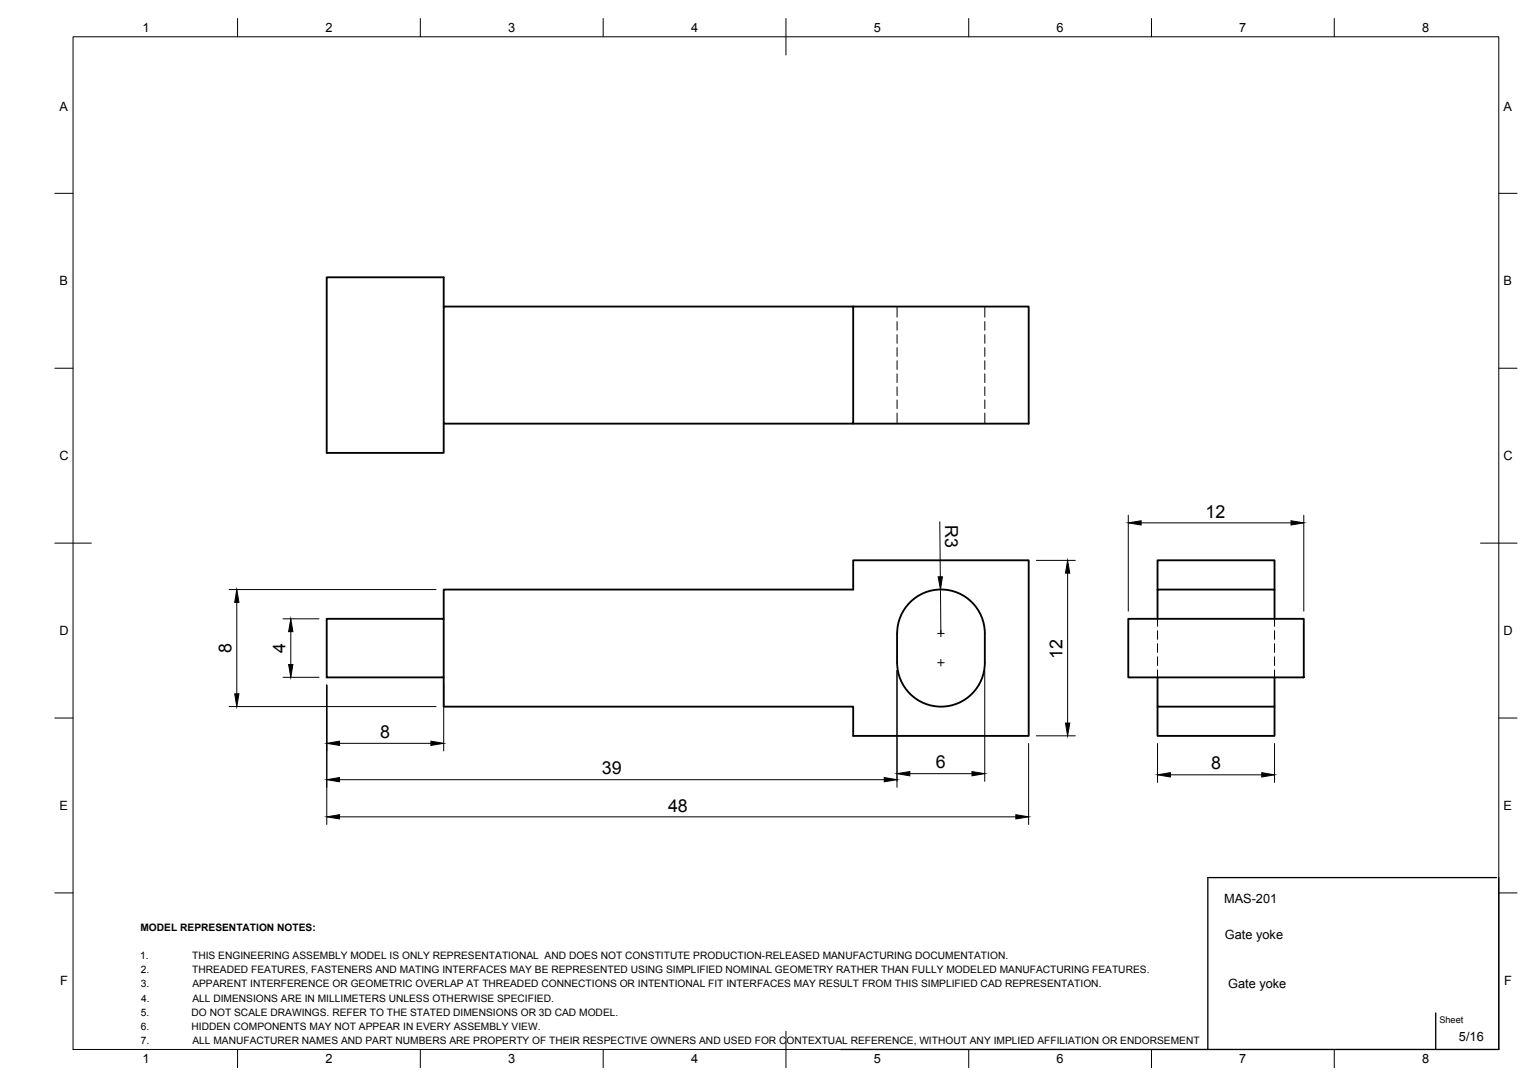
ISO-10303-21;
HEADER;
/* Generated by software containing ST-Developer
 * from STEP Tools, Inc. (www.steptools.com) 
 */

FILE_DESCRIPTION(
/* description */ ('Independent manual two-gate roller-track escapement for nominal30mm d
iameter20mm wide feed rollers. Opposed gates are driven by native capt
ured pin-slot loops with positive curved-slot travel stops at\X\B116de
g. Repeated gate/pin/washer/clip instances, adapted native common bear
ing families, full retaining lips and rotating polymer grip. External 
workpieces, gravity feeder/incline and mount anchors outside assembly.
 No powered-feed compatibility, impact, capacity, safety, force, wear 
or life rating.'),
/* implementation_level */ '2;1');

FILE_NAME(
/* name */ 'Gate yoke.step',
/* time_stamp */ '2026-11-08T18:43:23-08:00',
/* author */ (''),
/* organization */ (''),
/* preprocessor_version */ 'ST-DEVELOPER v20.2',
/* originating_system */ 'Autodesk Translation Framework v15.17.0.0',
/* authorisation */ '');

FILE_SCHEMA (('AUTOMOTIVE_DESIGN { 1 0 10303 214 3 1 1 }'));
ENDSEC;

DATA;
#10=MECHANICAL_DESIGN_GEOMETRIC_PRESENTATION_REPRESENTATION('',(#458),#19863);
#420=SHAPE_REPRESENTATION_RELATIONSHIP('SRR','None',#19938,#439);
#439=ADVANCED_BREP_SHAPE_REPRESENTATION('',(#477),#19847);
#458=STYLED_ITEM('',(#20041),#477);
#477=MANIFOLD_SOLID_BREP('Body1',#6427);
#774=LINE('',#15657,#1239);
#775=LINE('',#15659,#1240);
#776=LINE('',#15661,#1241);
#777=LINE('',#15662,#1242);
#778=LINE('',#15667,#1243);
#779=LINE('',#15671,#1244);
#780=LINE('',#15673,#1245);
#781=LINE('',#15674,#1246);
#782=LINE('',#15681,#1247);
#783=LINE('',#15683,#1248);
#784=LINE('',#15685,#1249);
#785=LINE('',#15686,#1250);
#786=LINE('',#15690,#1251);
#787=LINE('',#15692,#1252);
#788=LINE('',#15694,#1253);
#789=LINE('',#15695,#1254);
#790=LINE('',#15698,#1255);
#791=LINE('',#15700,#1256);
#792=LINE('',#15701,#1257);
#793=LINE('',#15703,#1258);
#794=LINE('',#15705,#1259);
#795=LINE('',#15706,#1260);
#796=LINE('',#15709,#1261);
#797=LINE('',#15710,#1262);
#798=LINE('',#15712,#1263);
#799=LINE('',#15713,#1264);
#800=LINE('',#15717,#1265);
#801=LINE('',#15719,#1266);
#802=LINE('',#15720,#1267);
#803=LINE('',#15723,#1268);
#804=LINE('',#15725,#1269);
#805=LINE('',#15726,#1270);
#806=LINE('',#15730,#1271);
#807=LINE('',#15731,#1272);
#808=LINE('',#15732,#1273);
#809=LINE('',#15736,#1274);
#810=LINE('',#15737,#1275);
#811=LINE('',#15738,#1276);
#812=LINE('',#15741,#1277);
#813=LINE('',#15743,#1278);
#814=LINE('',#15744,#1279);
#815=LINE('',#15748,#1280);
#816=LINE('',#15749,#1281);
#817=LINE('',#15751,#1282);
#818=LINE('',#15752,#1283);
#819=LINE('',#15755,#1284);
#820=LINE('',#15757,#1285);
#821=LINE('',#15758,#1286);
#822=LINE('',#15761,#1287);
#823=LINE('',#15762,#1288);
#824=LINE('',#15763,#1289);
#825=LINE('',#15765,#1290);
#1239=VECTOR('',#7968,10.);
#1240=VECTOR('',#7969,10.);
#1241=VECTOR('',#7970,10.);
#1242=VECTOR('',#7971,10.);
#1243=VECTOR('',#7976,10.);
#1244=VECTOR('',#7981,10.);
#1245=VECTOR('',#7982,10.);
#1246=VECTOR('',#7983,10.);
#1247=VECTOR('',#7992,10.);
#1248=VECTOR('',#7993,10.);
#1249=VECTOR('',#7994,10.);
#1250=VECTOR('',#7995,10.);
#1251=VECTOR('',#7998,10.);
#1252=VECTOR('',#7999,10.);
#1253=VECTOR('',#8000,10.);
#1254=VECTOR('',#8001,10.);
#1255=VECTOR('',#8004,10.);
#1256=VECTOR('',#8005,10.);
#1257=VECTOR('',#8006,10.);
#1258=VECTOR('',#8009,10.);
#1259=VECTOR('',#8010,10.);
#1260=VECTOR('',#8011,10.);
#1261=VECTOR('',#8014,10.);
#1262=VECTOR('',#8015,10.);
#1263=VECTOR('',#8018,10.);
#1264=VECTOR('',#8019,10.);
#1265=VECTOR('',#8024,10.);
#1266=VECTOR('',#8025,10.);
#1267=VECTOR('',#8026,10.);
#1268=VECTOR('',#8029,10.);
#1269=VECTOR('',#8030,10.);
#1270=VECTOR('',#8031,10.);
#1271=VECTOR('',#8034,10.);
#1272=VECTOR('',#8035,10.);
#1273=VECTOR('',#8036,10.);
#1274=VECTOR('',#8039,10.);
#1275=VECTOR('',#8040,10.);
#1276=VECTOR('',#8041,10.);
#1277=VECTOR('',#8044,10.);
#1278=VECTOR('',#8045,10.);
#1279=VECTOR('',#8046,10.);
#1280=VECTOR('',#8049,10.);
#1281=VECTOR('',#8050,10.);
#1282=VECTOR('',#8051,10.);
#1283=VECTOR('',#8052,10.);
#1284=VECTOR('',#8055,10.);
#1285=VECTOR('',#8056,10.);
#1286=VECTOR('',#8057,10.);
#1287=VECTOR('',#8060,10.);
#1288=VECTOR('',#8061,10.);
#1289=VECTOR('',#8062,10.);
#1290=VECTOR('',#8065,10.);
#1534=CYLINDRICAL_SURFACE('',#6901,3.);
#1535=CYLINDRICAL_SURFACE('',#6905,3.);
#1657=FACE_BOUND('',#2291,.T.);
#1658=FACE_BOUND('',#2294,.T.);
#1875=FACE_OUTER_BOUND('',#2274,.T.);
#1876=FACE_OUTER_BOUND('',#2275,.T.);
#1877=FACE_OUTER_BOUND('',#2276,.T.);
#1878=FACE_OUTER_BOUND('',#2277,.T.);
#1879=FACE_OUTER_BOUND('',#2278,.T.);
#1880=FACE_OUTER_BOUND('',#2279,.T.);
#1881=FACE_OUTER_BOUND('',#2280,.T.);
#1882=FACE_OUTER_BOUND('',#2281,.T.);
#1883=FACE_OUTER_BOUND('',#2282,.T.);
#1884=FACE_OUTER_BOUND('',#2283,.T.);
#1885=FACE_OUTER_BOUND('',#2284,.T.);
#1886=FACE_OUTER_BOUND('',#2285,.T.);
#1887=FACE_OUTER_BOUND('',#2286,.T.);
#1888=FACE_OUTER_BOUND('',#2287,.T.);
#1889=FACE_OUTER_BOUND('',#2288,.T.);
#1890=FACE_OUTER_BOUND('',#2289,.T.);
#1891=FACE_OUTER_BOUND('',#2290,.T.);
#1892=FACE_OUTER_BOUND('',#2292,.T.);
#1893=FACE_OUTER_BOUND('',#2293,.T.);
#1894=FACE_OUTER_BOUND('',#2295,.T.);
#1895=FACE_OUTER_BOUND('',#2296,.T.);
#1896=FACE_OUTER_BOUND('',#2297,.T.);
#2274=EDGE_LOOP('',(#5177,#5178,#5179,#5180));
#2275=EDGE_LOOP('',(#5181,#5182,#5183,#5184));
#2276=EDGE_LOOP('',(#5185,#5186,#5187,#5188));
#2277=EDGE_LOOP('',(#5189,#5190,#5191,#5192));
#2278=EDGE_LOOP('',(#5193,#5194,#5195,#5196));
#2279=EDGE_LOOP('',(#5197,#5198,#5199,#5200));
#2280=EDGE_LOOP('',(#5201,#5202,#5203,#5204));
#2281=EDGE_LOOP('',(#5205,#5206,#5207,#5208,#5209,#5210));
#2282=EDGE_LOOP('',(#5211,#5212,#5213,#5214));
#2283=EDGE_LOOP('',(#5215,#5216,#5217,#5218,#5219,#5220));
#2284=EDGE_LOOP('',(#5221,#5222,#5223,#5224));
#2285=EDGE_LOOP('',(#5225,#5226,#5227,#5228));
#2286=EDGE_LOOP('',(#5229,#5230,#5231,#5232));
#2287=EDGE_LOOP('',(#5233,#5234,#5235,#5236));
#2288=EDGE_LOOP('',(#5237,#5238,#5239,#5240));
#2289=EDGE_LOOP('',(#5241,#5242,#5243,#5244));
#2290=EDGE_LOOP('',(#5245,#5246,#5247,#5248,#5249,#5250,#5251,#5252,#5253,
#5254));
#2291=EDGE_LOOP('',(#5255,#5256,#5257,#5258));
#2292=EDGE_LOOP('',(#5259,#5260,#5261,#5262));
#2293=EDGE_LOOP('',(#5263,#5264,#5265,#5266,#5267,#5268,#5269,#5270,#5271,
#5272));
#2294=EDGE_LOOP('',(#5273,#5274,#5275,#5276));
#2295=EDGE_LOOP('',(#5277,#5278,#5279,#5280));
#2296=EDGE_LOOP('',(#5281,#5282,#5283,#5284));
#2297=EDGE_LOOP('',(#5285,#5286,#5287,#5288));
#2534=CIRCLE('',#6902,3.);
#2535=CIRCLE('',#6903,3.);
#2536=CIRCLE('',#6906,3.);
#2537=CIRCLE('',#6907,3.);
#2972=VERTEX_POINT('',#15655);
#2973=VERTEX_POINT('',#15656);
#2974=VERTEX_POINT('',#15658);
#2975=VERTEX_POINT('',#15660);
#2976=VERTEX_POINT('',#15664);
#2977=VERTEX_POINT('',#15666);
#2978=VERTEX_POINT('',#15670);
#2979=VERTEX_POINT('',#15672);
#2980=VERTEX_POINT('',#15679);
#2981=VERTEX_POINT('',#15680);
#2982=VERTEX_POINT('',#15682);
#2983=VERTEX_POINT('',#15684);
#2984=VERTEX_POINT('',#15688);
#2985=VERTEX_POINT('',#15689);
#2986=VERTEX_POINT('',#15691);
#2987=VERTEX_POINT('',#15693);
#2988=VERTEX_POINT('',#15697);
#2989=VERTEX_POINT('',#15699);
#2990=VERTEX_POINT('',#15704);
#2991=VERTEX_POINT('',#15708);
#2992=VERTEX_POINT('',#15716);
#2993=VERTEX_POINT('',#15718);
#2994=VERTEX_POINT('',#15722);
#2995=VERTEX_POINT('',#15724);
#2996=VERTEX_POINT('',#15728);
#2997=VERTEX_POINT('',#15729);
#2998=VERTEX_POINT('',#15734);
#2999=VERTEX_POINT('',#15735);
#3000=VERTEX_POINT('',#15740);
#3001=VERTEX_POINT('',#15742);
#3002=VERTEX_POINT('',#15746);
#3003=VERTEX_POINT('',#15747);
#3004=VERTEX_POINT('',#15750);
#3005=VERTEX_POINT('',#15754);
#3006=VERTEX_POINT('',#15756);
#3007=VERTEX_POINT('',#15760);
#3747=EDGE_CURVE('',#2972,#2973,#774,.T.);
#3748=EDGE_CURVE('',#2974,#2973,#775,.T.);
#3749=EDGE_CURVE('',#2974,#2975,#776,.T.);
#3750=EDGE_CURVE('',#2972,#2975,#777,.T.);
#3751=EDGE_CURVE('',#2976,#2974,#2534,.T.);
#3752=EDGE_CURVE('',#2976,#2977,#778,.T.);
#3753=EDGE_CURVE('',#2975,#2977,#2535,.T.);
#3754=EDGE_CURVE('',#2978,#2976,#779,.T.);
#3755=EDGE_CURVE('',#2978,#2979,#780,.T.);
#3756=EDGE_CURVE('',#2977,#2979,#781,.T.);
#3757=EDGE_CURVE('',#2973,#2978,#2536,.T.);
#3758=EDGE_CURVE('',#2979,#2972,#2537,.T.);
#3759=EDGE_CURVE('',#2980,#2981,#782,.T.);
#3760=EDGE_CURVE('',#2982,#2981,#783,.T.);
#3761=EDGE_CURVE('',#2983,#2982,#784,.T.);
#3762=EDGE_CURVE('',#2980,#2983,#785,.T.);
#3763=EDGE_CURVE('',#2984,#2985,#786,.T.);
#3764=EDGE_CURVE('',#2986,#2985,#787,.T.);
#3765=EDGE_CURVE('',#2987,#2986,#788,.T.);
#3766=EDGE_CURVE('',#2984,#2987,#789,.T.);
#3767=EDGE_CURVE('',#2986,#2988,#790,.T.);
#3768=EDGE_CURVE('',#2989,#2988,#791,.T.);
#3769=EDGE_CURVE('',#2987,#2989,#792,.T.);
#3770=EDGE_CURVE('',#2984,#2981,#793,.T.);
#3771=EDGE_CURVE('',#2990,#2989,#794,.T.);
#3772=EDGE_CURVE('',#2982,#2990,#795,.T.);
#3773=EDGE_CURVE('',#2991,#2990,#796,.T.);
#3774=EDGE_CURVE('',#2983,#2991,#797,.T.);
#3775=EDGE_CURVE('',#2980,#2985,#798,.T.);
#3776=EDGE_CURVE('',#2988,#2991,#799,.T.);
#3777=EDGE_CURVE('',#2985,#2992,#800,.T.);
#3778=EDGE_CURVE('',#2992,#2993,#801,.T.);
#3779=EDGE_CURVE('',#2993,#2980,#802,.T.);
#3780=EDGE_CURVE('',#2981,#2994,#803,.T.);
#3781=EDGE_CURVE('',#2994,#2995,#804,.T.);
#3782=EDGE_CURVE('',#2995,#2984,#805,.T.);
#3783=EDGE_CURVE('',#2996,#2997,#806,.T.);
#3784=EDGE_CURVE('',#2996,#2995,#807,.T.);
#3785=EDGE_CURVE('',#2997,#2994,#808,.T.);
#3786=EDGE_CURVE('',#2998,#2999,#809,.T.);
#3787=EDGE_CURVE('',#2998,#2993,#810,.T.);
#3788=EDGE_CURVE('',#2999,#2992,#811,.T.);
#3789=EDGE_CURVE('',#2999,#3000,#812,.T.);
#3790=EDGE_CURVE('',#3000,#3001,#813,.T.);
#3791=EDGE_CURVE('',#3001,#2998,#814,.T.);
#3792=EDGE_CURVE('',#3002,#3003,#815,.T.);
#3793=EDGE_CURVE('',#3003,#3000,#816,.T.);
#3794=EDGE_CURVE('',#3004,#2996,#817,.T.);
#3795=EDGE_CURVE('',#3002,#3004,#818,.T.);
#3796=EDGE_CURVE('',#3005,#3002,#819,.T.);
#3797=EDGE_CURVE('',#3006,#3004,#820,.T.);
#3798=EDGE_CURVE('',#3005,#3006,#821,.T.);
#3799=EDGE_CURVE('',#3007,#3005,#822,.T.);
#3800=EDGE_CURVE('',#2997,#3006,#823,.T.);
#3801=EDGE_CURVE('',#3007,#3001,#824,.T.);
#3802=EDGE_CURVE('',#3003,#3007,#825,.T.);
#5177=ORIENTED_EDGE('',*,*,#3747,.T.);
#5178=ORIENTED_EDGE('',*,*,#3748,.F.);
#5179=ORIENTED_EDGE('',*,*,#3749,.T.);
#5180=ORIENTED_EDGE('',*,*,#3750,.F.);
#5181=ORIENTED_EDGE('',*,*,#3749,.F.);
#5182=ORIENTED_EDGE('',*,*,#3751,.F.);
#5183=ORIENTED_EDGE('',*,*,#3752,.T.);
#5184=ORIENTED_EDGE('',*,*,#3753,.F.);
#5185=ORIENTED_EDGE('',*,*,#3752,.F.);
#5186=ORIENTED_EDGE('',*,*,#3754,.F.);
#5187=ORIENTED_EDGE('',*,*,#3755,.T.);
#5188=ORIENTED_EDGE('',*,*,#3756,.F.);
#5189=ORIENTED_EDGE('',*,*,#3755,.F.);
#5190=ORIENTED_EDGE('',*,*,#3757,.F.);
#5191=ORIENTED_EDGE('',*,*,#3747,.F.);
#5192=ORIENTED_EDGE('',*,*,#3758,.F.);
#5193=ORIENTED_EDGE('',*,*,#3759,.T.);
#5194=ORIENTED_EDGE('',*,*,#3760,.F.);
#5195=ORIENTED_EDGE('',*,*,#3761,.F.);
#5196=ORIENTED_EDGE('',*,*,#3762,.F.);
#5197=ORIENTED_EDGE('',*,*,#3763,.T.);
#5198=ORIENTED_EDGE('',*,*,#3764,.F.);
#5199=ORIENTED_EDGE('',*,*,#3765,.F.);
#5200=ORIENTED_EDGE('',*,*,#3766,.F.);
#5201=ORIENTED_EDGE('',*,*,#3765,.T.);
#5202=ORIENTED_EDGE('',*,*,#3767,.T.);
#5203=ORIENTED_EDGE('',*,*,#3768,.F.);
#5204=ORIENTED_EDGE('',*,*,#3769,.F.);
#5205=ORIENTED_EDGE('',*,*,#3760,.T.);
#5206=ORIENTED_EDGE('',*,*,#3770,.F.);
#5207=ORIENTED_EDGE('',*,*,#3766,.T.);
#5208=ORIENTED_EDGE('',*,*,#3769,.T.);
#5209=ORIENTED_EDGE('',*,*,#3771,.F.);
#5210=ORIENTED_EDGE('',*,*,#3772,.F.);
#5211=ORIENTED_EDGE('',*,*,#3761,.T.);
#5212=ORIENTED_EDGE('',*,*,#3772,.T.);
#5213=ORIENTED_EDGE('',*,*,#3773,.F.);
#5214=ORIENTED_EDGE('',*,*,#3774,.F.);
#5215=ORIENTED_EDGE('',*,*,#3764,.T.);
#5216=ORIENTED_EDGE('',*,*,#3775,.F.);
#5217=ORIENTED_EDGE('',*,*,#3762,.T.);
#5218=ORIENTED_EDGE('',*,*,#3774,.T.);
#5219=ORIENTED_EDGE('',*,*,#3776,.F.);
#5220=ORIENTED_EDGE('',*,*,#3767,.F.);
#5221=ORIENTED_EDGE('',*,*,#3776,.T.);
#5222=ORIENTED_EDGE('',*,*,#3773,.T.);
#5223=ORIENTED_EDGE('',*,*,#3771,.T.);
#5224=ORIENTED_EDGE('',*,*,#3768,.T.);
#5225=ORIENTED_EDGE('',*,*,#3775,.T.);
#5226=ORIENTED_EDGE('',*,*,#3777,.T.);
#5227=ORIENTED_EDGE('',*,*,#3778,.T.);
#5228=ORIENTED_EDGE('',*,*,#3779,.T.);
#5229=ORIENTED_EDGE('',*,*,#3770,.T.);
#5230=ORIENTED_EDGE('',*,*,#3780,.T.);
#5231=ORIENTED_EDGE('',*,*,#3781,.T.);
#5232=ORIENTED_EDGE('',*,*,#3782,.T.);
#5233=ORIENTED_EDGE('',*,*,#3783,.F.);
#5234=ORIENTED_EDGE('',*,*,#3784,.T.);
#5235=ORIENTED_EDGE('',*,*,#3781,.F.);
#5236=ORIENTED_EDGE('',*,*,#3785,.F.);
#5237=ORIENTED_EDGE('',*,*,#3786,.F.);
#5238=ORIENTED_EDGE('',*,*,#3787,.T.);
#5239=ORIENTED_EDGE('',*,*,#3778,.F.);
#5240=ORIENTED_EDGE('',*,*,#3788,.F.);
#5241=ORIENTED_EDGE('',*,*,#3786,.T.);
#5242=ORIENTED_EDGE('',*,*,#3789,.T.);
#5243=ORIENTED_EDGE('',*,*,#3790,.T.);
#5244=ORIENTED_EDGE('',*,*,#3791,.T.);
#5245=ORIENTED_EDGE('',*,*,#3792,.T.);
#5246=ORIENTED_EDGE('',*,*,#3793,.T.);
#5247=ORIENTED_EDGE('',*,*,#3789,.F.);
#5248=ORIENTED_EDGE('',*,*,#3788,.T.);
#5249=ORIENTED_EDGE('',*,*,#3777,.F.);
#5250=ORIENTED_EDGE('',*,*,#3763,.F.);
#5251=ORIENTED_EDGE('',*,*,#3782,.F.);
#5252=ORIENTED_EDGE('',*,*,#3784,.F.);
#5253=ORIENTED_EDGE('',*,*,#3794,.F.);
#5254=ORIENTED_EDGE('',*,*,#3795,.F.);
#5255=ORIENTED_EDGE('',*,*,#3750,.T.);
#5256=ORIENTED_EDGE('',*,*,#3753,.T.);
#5257=ORIENTED_EDGE('',*,*,#3756,.T.);
#5258=ORIENTED_EDGE('',*,*,#3758,.T.);
#5259=ORIENTED_EDGE('',*,*,#3796,.T.);
#5260=ORIENTED_EDGE('',*,*,#3795,.T.);
#5261=ORIENTED_EDGE('',*,*,#3797,.F.);
#5262=ORIENTED_EDGE('',*,*,#3798,.F.);
#5263=ORIENTED_EDGE('',*,*,#3799,.T.);
#5264=ORIENTED_EDGE('',*,*,#3798,.T.);
#5265=ORIENTED_EDGE('',*,*,#3800,.F.);
#5266=ORIENTED_EDGE('',*,*,#3785,.T.);
#5267=ORIENTED_EDGE('',*,*,#3780,.F.);
#5268=ORIENTED_EDGE('',*,*,#3759,.F.);
#5269=ORIENTED_EDGE('',*,*,#3779,.F.);
#5270=ORIENTED_EDGE('',*,*,#3787,.F.);
#5271=ORIENTED_EDGE('',*,*,#3791,.F.);
#5272=ORIENTED_EDGE('',*,*,#3801,.F.);
#5273=ORIENTED_EDGE('',*,*,#3748,.T.);
#5274=ORIENTED_EDGE('',*,*,#3757,.T.);
#5275=ORIENTED_EDGE('',*,*,#3754,.T.);
#5276=ORIENTED_EDGE('',*,*,#3751,.T.);
#5277=ORIENTED_EDGE('',*,*,#3802,.T.);
#5278=ORIENTED_EDGE('',*,*,#3801,.T.);
#5279=ORIENTED_EDGE('',*,*,#3790,.F.);
#5280=ORIENTED_EDGE('',*,*,#3793,.F.);
#5281=ORIENTED_EDGE('',*,*,#3783,.T.);
#5282=ORIENTED_EDGE('',*,*,#3800,.T.);
#5283=ORIENTED_EDGE('',*,*,#3797,.T.);
#5284=ORIENTED_EDGE('',*,*,#3794,.T.);
#5285=ORIENTED_EDGE('',*,*,#3802,.F.);
#5286=ORIENTED_EDGE('',*,*,#3792,.F.);
#5287=ORIENTED_EDGE('',*,*,#3796,.F.);
#5288=ORIENTED_EDGE('',*,*,#3799,.F.);
#5984=PLANE('',#6900);
#5985=PLANE('',#6904);
#5986=PLANE('',#6908);
#5987=PLANE('',#6909);
#5988=PLANE('',#6910);
#5989=PLANE('',#6911);
#5990=PLANE('',#6912);
#5991=PLANE('',#6913);
#5992=PLANE('',#6914);
#5993=PLANE('',#6915);
#5994=PLANE('',#6916);
#5995=PLANE('',#6917);
#5996=PLANE('',#6918);
#5997=PLANE('',#6919);
#5998=PLANE('',#6920);
#5999=PLANE('',#6921);
#6000=PLANE('',#6922);
#6001=PLANE('',#6923);
#6002=PLANE('',#6924);
#6003=PLANE('',#6925);
#6254=ADVANCED_FACE('',(#1875),#5984,.F.);
#6255=ADVANCED_FACE('',(#1876),#1534,.F.);
#6256=ADVANCED_FACE('',(#1877),#5985,.F.);
#6257=ADVANCED_FACE('',(#1878),#1535,.F.);
#6258=ADVANCED_FACE('',(#1879),#5986,.F.);
#6259=ADVANCED_FACE('',(#1880),#5987,.F.);
#6260=ADVANCED_FACE('',(#1881),#5988,.T.);
#6261=ADVANCED_FACE('',(#1882),#5989,.T.);
#6262=ADVANCED_FACE('',(#1883),#5990,.T.);
#6263=ADVANCED_FACE('',(#1884),#5991,.T.);
#6264=ADVANCED_FACE('',(#1885),#5992,.T.);
#6265=ADVANCED_FACE('',(#1886),#5993,.T.);
#6266=ADVANCED_FACE('',(#1887),#5994,.T.);
#6267=ADVANCED_FACE('',(#1888),#5995,.T.);
#6268=ADVANCED_FACE('',(#1889),#5996,.T.);
#6269=ADVANCED_FACE('',(#1890),#5997,.T.);
#6270=ADVANCED_FACE('',(#1891,#1657),#5998,.T.);
#6271=ADVANCED_FACE('',(#1892),#5999,.T.);
#6272=ADVANCED_FACE('',(#1893,#1658),#6000,.T.);
#6273=ADVANCED_FACE('',(#1894),#6001,.T.);
#6274=ADVANCED_FACE('',(#1895),#6002,.T.);
#6275=ADVANCED_FACE('',(#1896),#6003,.F.);
#6427=CLOSED_SHELL('',(#6254,#6255,#6256,#6257,#6258,#6259,#6260,#6261,
#6262,#6263,#6264,#6265,#6266,#6267,#6268,#6269,#6270,#6271,#6272,#6273,
#6274,#6275));
#6899=AXIS2_PLACEMENT_3D('',#15653,#7964,#7965);
#6900=AXIS2_PLACEMENT_3D('',#15654,#7966,#7967);
#6901=AXIS2_PLACEMENT_3D('',#15663,#7972,#7973);
#6902=AXIS2_PLACEMENT_3D('',#15665,#7974,#7975);
#6903=AXIS2_PLACEMENT_3D('',#15668,#7977,#7978);
#6904=AXIS2_PLACEMENT_3D('',#15669,#7979,#7980);
#6905=AXIS2_PLACEMENT_3D('',#15675,#7984,#7985);
#6906=AXIS2_PLACEMENT_3D('',#15676,#7986,#7987);
#6907=AXIS2_PLACEMENT_3D('',#15677,#7988,#7989);
#6908=AXIS2_PLACEMENT_3D('',#15678,#7990,#7991);
#6909=AXIS2_PLACEMENT_3D('',#15687,#7996,#7997);
#6910=AXIS2_PLACEMENT_3D('',#15696,#8002,#8003);
#6911=AXIS2_PLACEMENT_3D('',#15702,#8007,#8008);
#6912=AXIS2_PLACEMENT_3D('',#15707,#8012,#8013);
#6913=AXIS2_PLACEMENT_3D('',#15711,#8016,#8017);
#6914=AXIS2_PLACEMENT_3D('',#15714,#8020,#8021);
#6915=AXIS2_PLACEMENT_3D('',#15715,#8022,#8023);
#6916=AXIS2_PLACEMENT_3D('',#15721,#8027,#8028);
#6917=AXIS2_PLACEMENT_3D('',#15727,#8032,#8033);
#6918=AXIS2_PLACEMENT_3D('',#15733,#8037,#8038);
#6919=AXIS2_PLACEMENT_3D('',#15739,#8042,#8043);
#6920=AXIS2_PLACEMENT_3D('',#15745,#8047,#8048);
#6921=AXIS2_PLACEMENT_3D('',#15753,#8053,#8054);
#6922=AXIS2_PLACEMENT_3D('',#15759,#8058,#8059);
#6923=AXIS2_PLACEMENT_3D('',#15764,#8063,#8064);
#6924=AXIS2_PLACEMENT_3D('',#15766,#8066,#8067);
#6925=AXIS2_PLACEMENT_3D('',#15767,#8068,#8069);
#7964=DIRECTION('axis',(0.,0.,1.));
#7965=DIRECTION('refdir',(1.,0.,0.));
#7966=DIRECTION('center_axis',(0.,0.,1.));
#7967=DIRECTION('ref_axis',(1.,0.,0.));
#7968=DIRECTION('',(0.,-1.,0.));
#7969=DIRECTION('',(1.,0.,0.));
#7970=DIRECTION('',(0.,1.,0.));
#7971=DIRECTION('',(-1.,0.,0.));
#7972=DIRECTION('center_axis',(0.,1.,0.));
#7973=DIRECTION('ref_axis',(-9.25185853854298E-17,0.,-1.));
#7974=DIRECTION('center_axis',(0.,1.,0.));
#7975=DIRECTION('ref_axis',(-9.25185853854298E-17,0.,-1.));
#7976=DIRECTION('',(0.,1.,0.));
#7977=DIRECTION('center_axis',(0.,-1.,0.));
#7978=DIRECTION('ref_axis',(-9.25185853854298E-17,0.,-1.));
#7979=DIRECTION('center_axis',(0.,0.,-1.));
#7980=DIRECTION('ref_axis',(-1.,0.,0.));
#7981=DIRECTION('',(-1.,0.,0.));
#7982=DIRECTION('',(0.,1.,0.));
#7983=DIRECTION('',(1.,0.,0.));
#7984=DIRECTION('center_axis',(0.,1.,0.));
#7985=DIRECTION('ref_axis',(9.25185853854298E-17,0.,1.));
#7986=DIRECTION('center_axis',(0.,1.,0.));
#7987=DIRECTION('ref_axis',(9.25185853854298E-17,0.,1.));
#7988=DIRECTION('center_axis',(0.,-1.,0.));
#7989=DIRECTION('ref_axis',(9.25185853854298E-17,0.,1.));
#7990=DIRECTION('center_axis',(0.,0.,1.));
#7991=DIRECTION('ref_axis',(1.,0.,0.));
#7992=DIRECTION('',(1.,0.,0.));
#7993=DIRECTION('',(0.,1.,0.));
#7994=DIRECTION('',(1.,0.,0.));
#7995=DIRECTION('',(0.,-1.,0.));
#7996=DIRECTION('center_axis',(0.,0.,1.));
#7997=DIRECTION('ref_axis',(1.,0.,0.));
#7998=DIRECTION('',(-1.,0.,0.));
#7999=DIRECTION('',(0.,-1.,0.));
#8000=DIRECTION('',(-1.,0.,0.));
#8001=DIRECTION('',(0.,1.,0.));
#8002=DIRECTION('center_axis',(0.,1.,0.));
#8003=DIRECTION('ref_axis',(-1.,0.,0.));
#8004=DIRECTION('',(0.,0.,1.));
#8005=DIRECTION('',(-1.,0.,0.));
#8006=DIRECTION('',(0.,0.,1.));
#8007=DIRECTION('center_axis',(1.,0.,0.));
#8008=DIRECTION('ref_axis',(0.,1.,0.));
#8009=DIRECTION('',(0.,-1.,0.));
#8010=DIRECTION('',(0.,1.,0.));
#8011=DIRECTION('',(0.,0.,1.));
#8012=DIRECTION('center_axis',(0.,-1.,0.));
#8013=DIRECTION('ref_axis',(1.,0.,0.));
#8014=DIRECTION('',(1.,0.,0.));
#8015=DIRECTION('',(0.,0.,1.));
#8016=DIRECTION('center_axis',(-1.,0.,0.));
#8017=DIRECTION('ref_axis',(0.,-1.,0.));
#8018=DIRECTION('',(0.,1.,0.));
#8019=DIRECTION('',(0.,-1.,0.));
#8020=DIRECTION('center_axis',(0.,0.,1.));
#8021=DIRECTION('ref_axis',(1.,0.,0.));
#8022=DIRECTION('center_axis',(0.,0.,1.));
#8023=DIRECTION('ref_axis',(1.,0.,0.));
#8024=DIRECTION('',(-1.,0.,0.));
#8025=DIRECTION('',(0.,-1.,0.));
#8026=DIRECTION('',(1.,0.,0.));
#8027=DIRECTION('center_axis',(0.,0.,1.));
#8028=DIRECTION('ref_axis',(1.,0.,0.));
#8029=DIRECTION('',(1.,0.,0.));
#8030=DIRECTION('',(0.,1.,0.));
#8031=DIRECTION('',(-1.,0.,0.));
#8032=DIRECTION('center_axis',(1.,0.,0.));
#8033=DIRECTION('ref_axis',(0.,1.,0.));
#8034=DIRECTION('',(0.,-1.,0.));
#8035=DIRECTION('',(0.,0.,1.));
#8036=DIRECTION('',(0.,0.,1.));
#8037=DIRECTION('center_axis',(-1.,0.,0.));
#8038=DIRECTION('ref_axis',(0.,-1.,0.));
#8039=DIRECTION('',(0.,1.,0.));
#8040=DIRECTION('',(0.,0.,1.));
#8041=DIRECTION('',(0.,0.,1.));
#8042=DIRECTION('center_axis',(0.,0.,1.));
#8043=DIRECTION('ref_axis',(1.,0.,0.));
#8044=DIRECTION('',(-1.,0.,0.));
#8045=DIRECTION('',(0.,-1.,0.));
#8046=DIRECTION('',(1.,0.,0.));
#8047=DIRECTION('center_axis',(0.,1.,0.));
#8048=DIRECTION('ref_axis',(-1.,0.,0.));
#8049=DIRECTION('',(-1.,0.,0.));
#8050=DIRECTION('',(0.,0.,1.));
#8051=DIRECTION('',(-1.,0.,0.));
#8052=DIRECTION('',(0.,0.,1.));
#8053=DIRECTION('center_axis',(1.,0.,0.));
#8054=DIRECTION('ref_axis',(0.,1.,0.));
#8055=DIRECTION('',(0.,1.,0.));
#8056=DIRECTION('',(0.,1.,0.));
#8057=DIRECTION('',(0.,0.,1.));
#8058=DIRECTION('center_axis',(0.,-1.,0.));
#8059=DIRECTION('ref_axis',(1.,0.,0.));
#8060=DIRECTION('',(1.,0.,0.));
#8061=DIRECTION('',(1.,0.,0.));
#8062=DIRECTION('',(0.,0.,1.));
#8063=DIRECTION('center_axis',(-1.,0.,0.));
#8064=DIRECTION('ref_axis',(0.,-1.,0.));
#8065=DIRECTION('',(0.,-1.,0.));
#8066=DIRECTION('center_axis',(0.,0.,1.));
#8067=DIRECTION('ref_axis',(1.,0.,0.));
#8068=DIRECTION('center_axis',(0.,0.,1.));
#8069=DIRECTION('ref_axis',(1.,0.,0.));
#15653=CARTESIAN_POINT('',(0.,0.,0.));
#15654=CARTESIAN_POINT('Origin',(-1.,0.,-37.));
#15655=CARTESIAN_POINT('',(1.,4.,-37.));
#15656=CARTESIAN_POINT('',(1.,-4.,-37.));
#15657=CARTESIAN_POINT('',(1.,0.,-37.));
#15658=CARTESIAN_POINT('',(-1.,-4.,-37.));
#15659=CARTESIAN_POINT('',(-3.5,-4.,-37.));
#15660=CARTESIAN_POINT('',(-1.,4.,-37.));
#15661=CARTESIAN_POINT('',(-1.,0.,-37.));
#15662=CARTESIAN_POINT('',(2.5,4.,-37.));
#15663=CARTESIAN_POINT('Origin',(-1.,0.,-40.));
#15664=CARTESIAN_POINT('',(-1.,-4.,-43.));
#15665=CARTESIAN_POINT('Origin',(-1.,-4.,-40.));
#15666=CARTESIAN_POINT('',(-1.,4.,-43.));
#15667=CARTESIAN_POINT('',(-1.,0.,-43.));
#15668=CARTESIAN_POINT('Origin',(-1.,4.,-40.));
#15669=CARTESIAN_POINT('Origin',(1.,0.,-43.));
#15670=CARTESIAN_POINT('',(1.,-4.,-43.));
#15671=CARTESIAN_POINT('',(-2.5,-4.,-43.));
#15672=CARTESIAN_POINT('',(1.,4.,-43.));
#15673=CARTESIAN_POINT('',(1.,0.,-43.));
#15674=CARTESIAN_POINT('',(3.5,4.,-43.));
#15675=CARTESIAN_POINT('Origin',(1.,0.,-40.));
#15676=CARTESIAN_POINT('Origin',(1.,-4.,-40.));
#15677=CARTESIAN_POINT('Origin',(1.,4.,-40.));
#15678=CARTESIAN_POINT('Origin',(0.,0.,-6.));
#15679=CARTESIAN_POINT('',(-2.,-4.,-6.));
#15680=CARTESIAN_POINT('',(2.,-4.,-6.));
#15681=CARTESIAN_POINT('',(-4.,-4.,-6.));
#15682=CARTESIAN_POINT('',(2.,-6.,-6.));
#15683=CARTESIAN_POINT('',(2.,-6.,-6.));
#15684=CARTESIAN_POINT('',(-2.,-6.,-6.));
#15685=CARTESIAN_POINT('',(-2.,-6.,-6.));
#15686=CARTESIAN_POINT('',(-2.,6.,-6.));
#15687=CARTESIAN_POINT('Origin',(0.,0.,-6.));
#15688=CARTESIAN_POINT('',(2.,4.,-6.));
#15689=CARTESIAN_POINT('',(-2.,4.,-6.));
#15690=CARTESIAN_POINT('',(4.,4.,-6.));
#15691=CARTESIAN_POINT('',(-2.,6.,-6.));
#15692=CARTESIAN_POINT('',(-2.,6.,-6.));
#15693=CARTESIAN_POINT('',(2.,6.,-6.));
#15694=CARTESIAN_POINT('',(2.,6.,-6.));
#15695=CARTESIAN_POINT('',(2.,-6.,-6.));
#15696=CARTESIAN_POINT('Origin',(2.,6.,-6.));
#15697=CARTESIAN_POINT('',(-2.,6.,2.));
#15698=CARTESIAN_POINT('',(-2.,6.,-6.));
#15699=CARTESIAN_POINT('',(2.,6.,2.));
#15700=CARTESIAN_POINT('',(2.,6.,2.));
#15701=CARTESIAN_POINT('',(2.,6.,-6.));
#15702=CARTESIAN_POINT('Origin',(2.,-6.,-6.));
#15703=CARTESIAN_POINT('',(2.,-3.,-6.));
#15704=CARTESIAN_POINT('',(2.,-6.,2.));
#15705=CARTESIAN_POINT('',(2.,-6.,2.));
#15706=CARTESIAN_POINT('',(2.,-6.,-6.));
#15707=CARTESIAN_POINT('Origin',(-2.,-6.,-6.));
#15708=CARTESIAN_POINT('',(-2.,-6.,2.));
#15709=CARTESIAN_POINT('',(-2.,-6.,2.));
#15710=CARTESIAN_POINT('',(-2.,-6.,-6.));
#15711=CARTESIAN_POINT('Origin',(-2.,6.,-6.));
#15712=CARTESIAN_POINT('',(-2.,3.,-6.));
#15713=CARTESIAN_POINT('',(-2.,6.,2.));
#15714=CARTESIAN_POINT('Origin',(0.,0.,2.));
#15715=CARTESIAN_POINT('Origin',(0.,0.,-6.));
#15716=CARTESIAN_POINT('',(-4.,4.,-6.));
#15717=CARTESIAN_POINT('',(4.,4.,-6.));
#15718=CARTESIAN_POINT('',(-4.,-4.,-6.));
#15719=CARTESIAN_POINT('',(-4.,4.,-6.));
#15720=CARTESIAN_POINT('',(-4.,-4.,-6.));
#15721=CARTESIAN_POINT('Origin',(0.,0.,-6.));
#15722=CARTESIAN_POINT('',(4.,-4.,-6.));
#15723=CARTESIAN_POINT('',(-4.,-4.,-6.));
#15724=CARTESIAN_POINT('',(4.,4.,-6.));
#15725=CARTESIAN_POINT('',(4.,-4.,-6.));
#15726=CARTESIAN_POINT('',(4.,4.,-6.));
#15727=CARTESIAN_POINT('Origin',(4.,-4.,-34.));
#15728=CARTESIAN_POINT('',(4.,4.,-34.));
#15729=CARTESIAN_POINT('',(4.,-4.,-34.));
#15730=CARTESIAN_POINT('',(4.,-2.,-34.));
#15731=CARTESIAN_POINT('',(4.,4.,-34.));
#15732=CARTESIAN_POINT('',(4.,-4.,-34.));
#15733=CARTESIAN_POINT('Origin',(-4.,4.,-34.));
#15734=CARTESIAN_POINT('',(-4.,-4.,-34.));
#15735=CARTESIAN_POINT('',(-4.,4.,-34.));
#15736=CARTESIAN_POINT('',(-4.,2.,-34.));
#15737=CARTESIAN_POINT('',(-4.,-4.,-34.));
#15738=CARTESIAN_POINT('',(-4.,4.,-34.));
#15739=CARTESIAN_POINT('Origin',(0.,0.,-34.));
#15740=CARTESIAN_POINT('',(-6.,4.,-34.));
#15741=CARTESIAN_POINT('',(6.,4.,-34.));
#15742=CARTESIAN_POINT('',(-6.,-4.,-34.));
#15743=CARTESIAN_POINT('',(-6.,4.,-34.));
#15744=CARTESIAN_POINT('',(-6.,-4.,-34.));
#15745=CARTESIAN_POINT('Origin',(6.,4.,-46.));
#15746=CARTESIAN_POINT('',(6.,4.,-46.));
#15747=CARTESIAN_POINT('',(-6.,4.,-46.));
#15748=CARTESIAN_POINT('',(6.,4.,-46.));
#15749=CARTESIAN_POINT('',(-6.,4.,-46.));
#15750=CARTESIAN_POINT('',(6.,4.,-34.));
#15751=CARTESIAN_POINT('',(6.,4.,-34.));
#15752=CARTESIAN_POINT('',(6.,4.,-46.));
#15753=CARTESIAN_POINT('Origin',(6.,-4.,-46.));
#15754=CARTESIAN_POINT('',(6.,-4.,-46.));
#15755=CARTESIAN_POINT('',(6.,-4.,-46.));
#15756=CARTESIAN_POINT('',(6.,-4.,-34.));
#15757=CARTESIAN_POINT('',(6.,-4.,-34.));
#15758=CARTESIAN_POINT('',(6.,-4.,-46.));
#15759=CARTESIAN_POINT('Origin',(-6.,-4.,-46.));
#15760=CARTESIAN_POINT('',(-6.,-4.,-46.));
#15761=CARTESIAN_POINT('',(-6.,-4.,-46.));
#15762=CARTESIAN_POINT('',(-6.,-4.,-34.));
#15763=CARTESIAN_POINT('',(-6.,-4.,-46.));
#15764=CARTESIAN_POINT('Origin',(-6.,4.,-46.));
#15765=CARTESIAN_POINT('',(-6.,4.,-46.));
#15766=CARTESIAN_POINT('Origin',(0.,0.,-34.));
#15767=CARTESIAN_POINT('Origin',(0.,0.,-46.));
#19826=UNCERTAINTY_MEASURE_WITH_UNIT(LENGTH_MEASURE(0.01),#19864,
'DISTANCE_ACCURACY_VALUE',
'Maximum model space distance between geometric entities at asserted c
onnectivities');
#19842=UNCERTAINTY_MEASURE_WITH_UNIT(LENGTH_MEASURE(0.01),#19864,
'DISTANCE_ACCURACY_VALUE',
'Maximum model space distance between geometric entities at asserted c
onnectivities');
#19847=(
GEOMETRIC_REPRESENTATION_CONTEXT(3)
GLOBAL_UNCERTAINTY_ASSIGNED_CONTEXT((#19826))
GLOBAL_UNIT_ASSIGNED_CONTEXT((#19864,#19866,#19867))
REPRESENTATION_CONTEXT('','3D')
);
#19863=(
GEOMETRIC_REPRESENTATION_CONTEXT(3)
GLOBAL_UNCERTAINTY_ASSIGNED_CONTEXT((#19842))
GLOBAL_UNIT_ASSIGNED_CONTEXT((#19864,#19866,#19867))
REPRESENTATION_CONTEXT('','3D')
);
#19864=(
LENGTH_UNIT()
NAMED_UNIT(*)
SI_UNIT(.MILLI.,.METRE.)
);
#19866=(
NAMED_UNIT(*)
PLANE_ANGLE_UNIT()
SI_UNIT($,.RADIAN.)
);
#19867=(
NAMED_UNIT(*)
SI_UNIT($,.STERADIAN.)
SOLID_ANGLE_UNIT()
);
#19872=SHAPE_DEFINITION_REPRESENTATION(#19892,#19938);
#19892=PRODUCT_DEFINITION_SHAPE('',$,#19959);
#19938=SHAPE_REPRESENTATION('',(#6899),#19847);
#19954=PRODUCT_DEFINITION_CONTEXT('part definition',#20016,'design');
#19959=PRODUCT_DEFINITION('Gate yoke','Gate yoke',#19979,#19954);
#19979=PRODUCT_DEFINITION_FORMATION('',$,#20022);
#20016=APPLICATION_CONTEXT(
'Core Data for Automotive Mechanical Design Process');
#20017=PRODUCT_CONTEXT('part definition',#20016,'mechanical');
#20022=PRODUCT('Gate yoke','Gate yoke',$,(#20017));
#20041=PRESENTATION_STYLE_ASSIGNMENT((#20048));
#20048=SURFACE_STYLE_USAGE(.BOTH.,#20055);
#20055=SURFACE_SIDE_STYLE('',(#20062));
#20062=SURFACE_STYLE_FILL_AREA(#20069);
#20069=FILL_AREA_STYLE('Sky blue',(#20076));
#20076=FILL_AREA_STYLE_COLOUR('Sky blue',#20083);
#20083=COLOUR_RGB('Sky blue',0.317647058823529,0.686274509803922,0.890196078431372);
ENDSEC;
END-ISO-10303-21;
